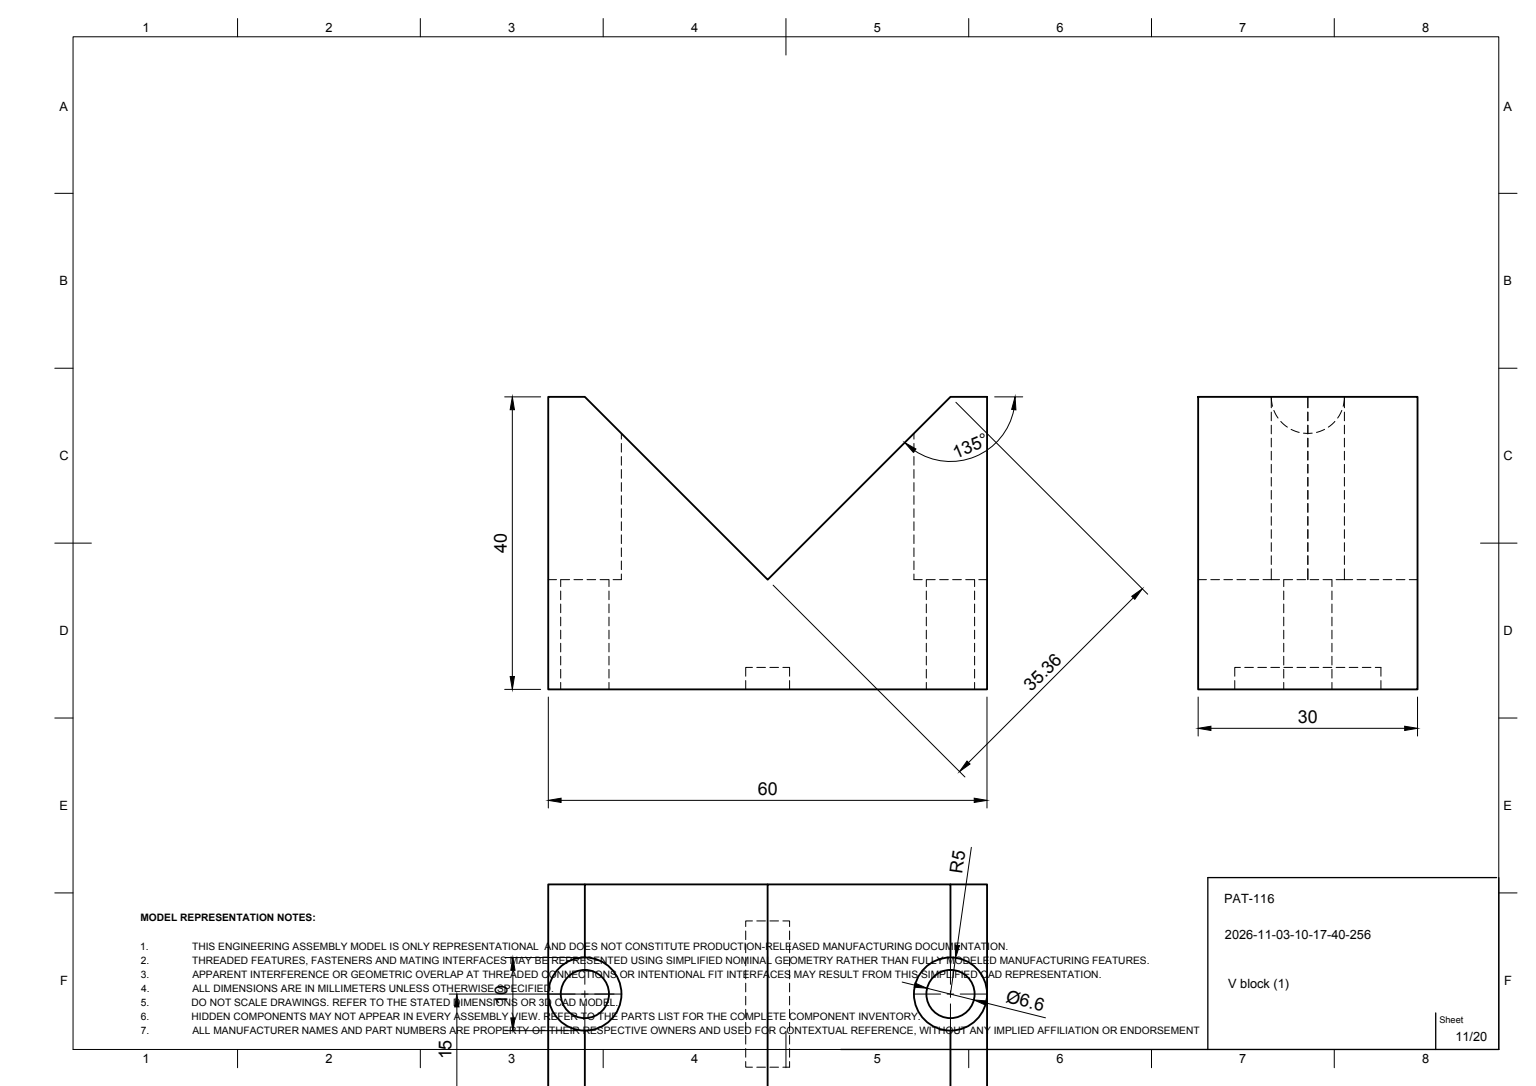
ISO-10303-21;
HEADER;
/* Generated by software containing ST-Developer
 * from STEP Tools, Inc. (www.steptools.com) 
 */

FILE_DESCRIPTION(
/* description */ ('V-block with clamp strap'),
/* implementation_level */ '2;1');

FILE_NAME(
/* name */ 'V block (1).step',
/* time_stamp */ '2026-10-27T10:50:53-07:00',
/* author */ (''),
/* organization */ (''),
/* preprocessor_version */ 'ST-DEVELOPER v20.2',
/* originating_system */ 'Autodesk Translation Framework v15.17.0.0',
/* authorisation */ '');

FILE_SCHEMA (('AUTOMOTIVE_DESIGN { 1 0 10303 214 3 1 1 }'));
ENDSEC;

DATA;
#10=MECHANICAL_DESIGN_GEOMETRIC_PRESENTATION_REPRESENTATION('',(#272),#7344);
#222=ELLIPSE('',#4545,0.707106781186547,0.5);
#223=ELLIPSE('',#4557,0.707106781186547,0.5);
#230=SHAPE_REPRESENTATION_RELATIONSHIP('SRR','None',#7448,#251);
#251=ADVANCED_BREP_SHAPE_REPRESENTATION('',(#293),#7327);
#272=STYLED_ITEM('',(#7610),#293);
#293=MANIFOLD_SOLID_BREP('Body1',#4154);
#344=FACE_BOUND('',#930,.T.);
#345=FACE_BOUND('',#933,.T.);
#346=FACE_BOUND('',#947,.T.);
#347=FACE_BOUND('',#948,.T.);
#348=FACE_BOUND('',#949,.T.);
#420=CIRCLE('',#4540,0.5);
#421=CIRCLE('',#4541,0.5);
#422=CIRCLE('',#4543,0.5);
#423=CIRCLE('',#4544,0.5);
#424=CIRCLE('',#4552,0.5);
#425=CIRCLE('',#4553,0.5);
#426=CIRCLE('',#4555,0.33);
#427=CIRCLE('',#4558,0.5);
#428=CIRCLE('',#4559,0.5);
#429=CIRCLE('',#4561,0.33);
#430=CIRCLE('',#4567,0.33);
#431=CIRCLE('',#4569,0.33);
#527=CYLINDRICAL_SURFACE('',#4539,0.5);
#528=CYLINDRICAL_SURFACE('',#4542,0.5);
#529=CYLINDRICAL_SURFACE('',#4551,0.5);
#530=CYLINDRICAL_SURFACE('',#4556,0.5);
#531=CYLINDRICAL_SURFACE('',#4566,0.33);
#532=CYLINDRICAL_SURFACE('',#4568,0.33);
#642=FACE_OUTER_BOUND('',#921,.T.);
#643=FACE_OUTER_BOUND('',#922,.T.);
#644=FACE_OUTER_BOUND('',#923,.T.);
#645=FACE_OUTER_BOUND('',#924,.T.);
#646=FACE_OUTER_BOUND('',#925,.T.);
#647=FACE_OUTER_BOUND('',#926,.T.);
#648=FACE_OUTER_BOUND('',#927,.T.);
#649=FACE_OUTER_BOUND('',#928,.T.);
#650=FACE_OUTER_BOUND('',#929,.T.);
#651=FACE_OUTER_BOUND('',#931,.T.);
#652=FACE_OUTER_BOUND('',#932,.T.);
#653=FACE_OUTER_BOUND('',#934,.T.);
#654=FACE_OUTER_BOUND('',#935,.T.);
#655=FACE_OUTER_BOUND('',#936,.T.);
#656=FACE_OUTER_BOUND('',#937,.T.);
#657=FACE_OUTER_BOUND('',#938,.T.);
#658=FACE_OUTER_BOUND('',#939,.T.);
#659=FACE_OUTER_BOUND('',#940,.T.);
#660=FACE_OUTER_BOUND('',#941,.T.);
#661=FACE_OUTER_BOUND('',#942,.T.);
#662=FACE_OUTER_BOUND('',#943,.T.);
#663=FACE_OUTER_BOUND('',#944,.T.);
#664=FACE_OUTER_BOUND('',#945,.T.);
#665=FACE_OUTER_BOUND('',#946,.T.);
#921=EDGE_LOOP('',(#3078,#3079,#3080,#3081));
#922=EDGE_LOOP('',(#3082,#3083,#3084,#3085,#3086));
#923=EDGE_LOOP('',(#3087,#3088,#3089,#3090));
#924=EDGE_LOOP('',(#3091,#3092,#3093,#3094));
#925=EDGE_LOOP('',(#3095,#3096,#3097,#3098));
#926=EDGE_LOOP('',(#3099,#3100,#3101,#3102));
#927=EDGE_LOOP('',(#3103,#3104,#3105,#3106));
#928=EDGE_LOOP('',(#3107,#3108,#3109,#3110));
#929=EDGE_LOOP('',(#3111,#3112));
#930=EDGE_LOOP('',(#3113));
#931=EDGE_LOOP('',(#3114,#3115,#3116,#3117,#3118));
#932=EDGE_LOOP('',(#3119,#3120));
#933=EDGE_LOOP('',(#3121));
#934=EDGE_LOOP('',(#3122,#3123,#3124,#3125,#3126,#3127));
#935=EDGE_LOOP('',(#3128,#3129,#3130,#3131));
#936=EDGE_LOOP('',(#3132,#3133,#3134,#3135,#3136,#3137));
#937=EDGE_LOOP('',(#3138,#3139,#3140,#3141));
#938=EDGE_LOOP('',(#3142,#3143,#3144,#3145));
#939=EDGE_LOOP('',(#3146,#3147,#3148,#3149));
#940=EDGE_LOOP('',(#3150,#3151,#3152,#3153));
#941=EDGE_LOOP('',(#3154,#3155,#3156,#3157));
#942=EDGE_LOOP('',(#3158,#3159,#3160,#3161,#3162,#3163,#3164));
#943=EDGE_LOOP('',(#3165,#3166,#3167,#3168,#3169,#3170,#3171));
#944=EDGE_LOOP('',(#3172,#3173,#3174,#3175,#3176,#3177,#3178));
#945=EDGE_LOOP('',(#3179,#3180,#3181,#3182,#3183,#3184,#3185));
#946=EDGE_LOOP('',(#3186,#3187,#3188,#3189));
#947=EDGE_LOOP('',(#3190,#3191,#3192,#3193));
#948=EDGE_LOOP('',(#3194));
#949=EDGE_LOOP('',(#3195));
#1258=LINE('',#6493,#1623);
#1259=LINE('',#6497,#1624);
#1260=LINE('',#6502,#1625);
#1261=LINE('',#6506,#1626);
#1262=LINE('',#6513,#1627);
#1263=LINE('',#6515,#1628);
#1264=LINE('',#6517,#1629);
#1265=LINE('',#6518,#1630);
#1266=LINE('',#6521,#1631);
#1267=LINE('',#6523,#1632);
#1268=LINE('',#6524,#1633);
#1269=LINE('',#6527,#1634);
#1270=LINE('',#6529,#1635);
#1271=LINE('',#6530,#1636);
#1272=LINE('',#6532,#1637);
#1273=LINE('',#6533,#1638);
#1274=LINE('',#6537,#1639);
#1275=LINE('',#6546,#1640);
#1276=LINE('',#6553,#1641);
#1277=LINE('',#6555,#1642);
#1278=LINE('',#6557,#1643);
#1279=LINE('',#6559,#1644);
#1280=LINE('',#6560,#1645);
#1281=LINE('',#6563,#1646);
#1282=LINE('',#6564,#1647);
#1283=LINE('',#6567,#1648);
#1284=LINE('',#6568,#1649);
#1285=LINE('',#6570,#1650);
#1286=LINE('',#6571,#1651);
#1287=LINE('',#6574,#1652);
#1288=LINE('',#6575,#1653);
#1289=LINE('',#6579,#1654);
#1290=LINE('',#6583,#1655);
#1291=LINE('',#6586,#1656);
#1292=LINE('',#6587,#1657);
#1293=LINE('',#6590,#1658);
#1294=LINE('',#6591,#1659);
#1295=LINE('',#6594,#1660);
#1296=LINE('',#6596,#1661);
#1297=LINE('',#6597,#1662);
#1298=LINE('',#6600,#1663);
#1299=LINE('',#6601,#1664);
#1300=LINE('',#6604,#1665);
#1301=LINE('',#6605,#1666);
#1302=LINE('',#6607,#1667);
#1623=VECTOR('',#5260,0.5);
#1624=VECTOR('',#5263,1.);
#1625=VECTOR('',#5268,0.5);
#1626=VECTOR('',#5271,1.);
#1627=VECTOR('',#5278,1.);
#1628=VECTOR('',#5279,1.);
#1629=VECTOR('',#5280,1.);
#1630=VECTOR('',#5281,1.);
#1631=VECTOR('',#5284,1.);
#1632=VECTOR('',#5285,1.);
#1633=VECTOR('',#5286,1.);
#1634=VECTOR('',#5289,1.);
#1635=VECTOR('',#5290,1.);
#1636=VECTOR('',#5291,1.);
#1637=VECTOR('',#5294,1.);
#1638=VECTOR('',#5295,1.);
#1639=VECTOR('',#5302,1.);
#1640=VECTOR('',#5315,1.);
#1641=VECTOR('',#5324,1.);
#1642=VECTOR('',#5325,1.);
#1643=VECTOR('',#5326,1.);
#1644=VECTOR('',#5327,1.);
#1645=VECTOR('',#5328,1.);
#1646=VECTOR('',#5331,1.);
#1647=VECTOR('',#5332,1.);
#1648=VECTOR('',#5335,1.);
#1649=VECTOR('',#5336,1.);
#1650=VECTOR('',#5337,1.);
#1651=VECTOR('',#5338,1.);
#1652=VECTOR('',#5341,1.);
#1653=VECTOR('',#5342,1.);
#1654=VECTOR('',#5347,0.33);
#1655=VECTOR('',#5352,0.33);
#1656=VECTOR('',#5355,1.);
#1657=VECTOR('',#5356,1.);
#1658=VECTOR('',#5359,1.);
#1659=VECTOR('',#5360,1.);
#1660=VECTOR('',#5363,1.);
#1661=VECTOR('',#5364,1.);
#1662=VECTOR('',#5365,1.);
#1663=VECTOR('',#5368,1.);
#1664=VECTOR('',#5369,1.);
#1665=VECTOR('',#5372,1.);
#1666=VECTOR('',#5373,1.);
#1667=VECTOR('',#5376,1.);
#1967=VERTEX_POINT('',#6491);
#1968=VERTEX_POINT('',#6492);
#1969=VERTEX_POINT('',#6494);
#1970=VERTEX_POINT('',#6496);
#1971=VERTEX_POINT('',#6500);
#1972=VERTEX_POINT('',#6501);
#1973=VERTEX_POINT('',#6503);
#1974=VERTEX_POINT('',#6505);
#1975=VERTEX_POINT('',#6507);
#1976=VERTEX_POINT('',#6511);
#1977=VERTEX_POINT('',#6512);
#1978=VERTEX_POINT('',#6514);
#1979=VERTEX_POINT('',#6516);
#1980=VERTEX_POINT('',#6520);
#1981=VERTEX_POINT('',#6522);
#1982=VERTEX_POINT('',#6526);
#1983=VERTEX_POINT('',#6528);
#1984=VERTEX_POINT('',#6540);
#1985=VERTEX_POINT('',#6543);
#1986=VERTEX_POINT('',#6549);
#1987=VERTEX_POINT('',#6552);
#1988=VERTEX_POINT('',#6554);
#1989=VERTEX_POINT('',#6556);
#1990=VERTEX_POINT('',#6558);
#1991=VERTEX_POINT('',#6562);
#1992=VERTEX_POINT('',#6566);
#1993=VERTEX_POINT('',#6569);
#1994=VERTEX_POINT('',#6573);
#1995=VERTEX_POINT('',#6577);
#1996=VERTEX_POINT('',#6581);
#1997=VERTEX_POINT('',#6585);
#1998=VERTEX_POINT('',#6589);
#1999=VERTEX_POINT('',#6593);
#2000=VERTEX_POINT('',#6595);
#2001=VERTEX_POINT('',#6599);
#2002=VERTEX_POINT('',#6603);
#2365=EDGE_CURVE('',#1967,#1968,#1258,.T.);
#2366=EDGE_CURVE('',#1969,#1967,#420,.T.);
#2367=EDGE_CURVE('',#1969,#1970,#1259,.T.);
#2368=EDGE_CURVE('',#1968,#1970,#421,.T.);
#2369=EDGE_CURVE('',#1971,#1972,#1260,.T.);
#2370=EDGE_CURVE('',#1973,#1971,#422,.T.);
#2371=EDGE_CURVE('',#1973,#1974,#1261,.T.);
#2372=EDGE_CURVE('',#1975,#1974,#423,.T.);
#2373=EDGE_CURVE('',#1972,#1975,#222,.T.);
#2374=EDGE_CURVE('',#1976,#1977,#1262,.T.);
#2375=EDGE_CURVE('',#1976,#1978,#1263,.T.);
#2376=EDGE_CURVE('',#1978,#1979,#1264,.T.);
#2377=EDGE_CURVE('',#1977,#1979,#1265,.T.);
#2378=EDGE_CURVE('',#1977,#1980,#1266,.T.);
#2379=EDGE_CURVE('',#1979,#1981,#1267,.T.);
#2380=EDGE_CURVE('',#1980,#1981,#1268,.T.);
#2381=EDGE_CURVE('',#1980,#1982,#1269,.T.);
#2382=EDGE_CURVE('',#1981,#1983,#1270,.T.);
#2383=EDGE_CURVE('',#1982,#1983,#1271,.T.);
#2384=EDGE_CURVE('',#1982,#1976,#1272,.T.);
#2385=EDGE_CURVE('',#1983,#1978,#1273,.T.);
#2386=EDGE_CURVE('',#1974,#1972,#424,.T.);
#2387=EDGE_CURVE('',#1973,#1974,#1274,.T.);
#2388=EDGE_CURVE('',#1971,#1973,#425,.T.);
#2389=EDGE_CURVE('',#1984,#1984,#426,.T.);
#2390=EDGE_CURVE('',#1985,#1968,#223,.T.);
#2391=EDGE_CURVE('',#1970,#1985,#427,.T.);
#2392=EDGE_CURVE('',#1969,#1970,#1275,.T.);
#2393=EDGE_CURVE('',#1967,#1969,#428,.T.);
#2394=EDGE_CURVE('',#1986,#1986,#429,.T.);
#2395=EDGE_CURVE('',#1987,#1975,#1276,.T.);
#2396=EDGE_CURVE('',#1988,#1987,#1277,.T.);
#2397=EDGE_CURVE('',#1989,#1988,#1278,.T.);
#2398=EDGE_CURVE('',#1990,#1989,#1279,.T.);
#2399=EDGE_CURVE('',#1972,#1990,#1280,.T.);
#2400=EDGE_CURVE('',#1974,#1991,#1281,.T.);
#2401=EDGE_CURVE('',#1991,#1987,#1282,.T.);
#2402=EDGE_CURVE('',#1992,#1968,#1283,.T.);
#2403=EDGE_CURVE('',#1989,#1992,#1284,.T.);
#2404=EDGE_CURVE('',#1993,#1988,#1285,.T.);
#2405=EDGE_CURVE('',#1985,#1993,#1286,.T.);
#2406=EDGE_CURVE('',#1970,#1994,#1287,.T.);
#2407=EDGE_CURVE('',#1994,#1992,#1288,.T.);
#2408=EDGE_CURVE('',#1995,#1995,#430,.T.);
#2409=EDGE_CURVE('',#1995,#1984,#1289,.T.);
#2410=EDGE_CURVE('',#1996,#1996,#431,.T.);
#2411=EDGE_CURVE('',#1996,#1986,#1290,.T.);
#2412=EDGE_CURVE('',#1990,#1997,#1291,.T.);
#2413=EDGE_CURVE('',#1997,#1974,#1292,.T.);
#2414=EDGE_CURVE('',#1993,#1998,#1293,.T.);
#2415=EDGE_CURVE('',#1998,#1970,#1294,.T.);
#2416=EDGE_CURVE('',#1999,#1994,#1295,.T.);
#2417=EDGE_CURVE('',#1999,#2000,#1296,.T.);
#2418=EDGE_CURVE('',#2000,#1997,#1297,.T.);
#2419=EDGE_CURVE('',#2001,#1999,#1298,.T.);
#2420=EDGE_CURVE('',#2001,#1998,#1299,.T.);
#2421=EDGE_CURVE('',#2002,#1991,#1300,.T.);
#2422=EDGE_CURVE('',#2002,#2001,#1301,.T.);
#2423=EDGE_CURVE('',#2000,#2002,#1302,.T.);
#3078=ORIENTED_EDGE('',*,*,#2365,.F.);
#3079=ORIENTED_EDGE('',*,*,#2366,.F.);
#3080=ORIENTED_EDGE('',*,*,#2367,.T.);
#3081=ORIENTED_EDGE('',*,*,#2368,.F.);
#3082=ORIENTED_EDGE('',*,*,#2369,.F.);
#3083=ORIENTED_EDGE('',*,*,#2370,.F.);
#3084=ORIENTED_EDGE('',*,*,#2371,.T.);
#3085=ORIENTED_EDGE('',*,*,#2372,.F.);
#3086=ORIENTED_EDGE('',*,*,#2373,.F.);
#3087=ORIENTED_EDGE('',*,*,#2374,.F.);
#3088=ORIENTED_EDGE('',*,*,#2375,.T.);
#3089=ORIENTED_EDGE('',*,*,#2376,.T.);
#3090=ORIENTED_EDGE('',*,*,#2377,.F.);
#3091=ORIENTED_EDGE('',*,*,#2378,.F.);
#3092=ORIENTED_EDGE('',*,*,#2377,.T.);
#3093=ORIENTED_EDGE('',*,*,#2379,.T.);
#3094=ORIENTED_EDGE('',*,*,#2380,.F.);
#3095=ORIENTED_EDGE('',*,*,#2381,.F.);
#3096=ORIENTED_EDGE('',*,*,#2380,.T.);
#3097=ORIENTED_EDGE('',*,*,#2382,.T.);
#3098=ORIENTED_EDGE('',*,*,#2383,.F.);
#3099=ORIENTED_EDGE('',*,*,#2384,.F.);
#3100=ORIENTED_EDGE('',*,*,#2383,.T.);
#3101=ORIENTED_EDGE('',*,*,#2385,.T.);
#3102=ORIENTED_EDGE('',*,*,#2375,.F.);
#3103=ORIENTED_EDGE('',*,*,#2385,.F.);
#3104=ORIENTED_EDGE('',*,*,#2382,.F.);
#3105=ORIENTED_EDGE('',*,*,#2379,.F.);
#3106=ORIENTED_EDGE('',*,*,#2376,.F.);
#3107=ORIENTED_EDGE('',*,*,#2369,.T.);
#3108=ORIENTED_EDGE('',*,*,#2386,.F.);
#3109=ORIENTED_EDGE('',*,*,#2387,.F.);
#3110=ORIENTED_EDGE('',*,*,#2388,.F.);
#3111=ORIENTED_EDGE('',*,*,#2370,.T.);
#3112=ORIENTED_EDGE('',*,*,#2388,.T.);
#3113=ORIENTED_EDGE('',*,*,#2389,.F.);
#3114=ORIENTED_EDGE('',*,*,#2365,.T.);
#3115=ORIENTED_EDGE('',*,*,#2390,.F.);
#3116=ORIENTED_EDGE('',*,*,#2391,.F.);
#3117=ORIENTED_EDGE('',*,*,#2392,.F.);
#3118=ORIENTED_EDGE('',*,*,#2393,.F.);
#3119=ORIENTED_EDGE('',*,*,#2366,.T.);
#3120=ORIENTED_EDGE('',*,*,#2393,.T.);
#3121=ORIENTED_EDGE('',*,*,#2394,.F.);
#3122=ORIENTED_EDGE('',*,*,#2373,.T.);
#3123=ORIENTED_EDGE('',*,*,#2395,.F.);
#3124=ORIENTED_EDGE('',*,*,#2396,.F.);
#3125=ORIENTED_EDGE('',*,*,#2397,.F.);
#3126=ORIENTED_EDGE('',*,*,#2398,.F.);
#3127=ORIENTED_EDGE('',*,*,#2399,.F.);
#3128=ORIENTED_EDGE('',*,*,#2372,.T.);
#3129=ORIENTED_EDGE('',*,*,#2400,.T.);
#3130=ORIENTED_EDGE('',*,*,#2401,.T.);
#3131=ORIENTED_EDGE('',*,*,#2395,.T.);
#3132=ORIENTED_EDGE('',*,*,#2390,.T.);
#3133=ORIENTED_EDGE('',*,*,#2402,.F.);
#3134=ORIENTED_EDGE('',*,*,#2403,.F.);
#3135=ORIENTED_EDGE('',*,*,#2397,.T.);
#3136=ORIENTED_EDGE('',*,*,#2404,.F.);
#3137=ORIENTED_EDGE('',*,*,#2405,.F.);
#3138=ORIENTED_EDGE('',*,*,#2368,.T.);
#3139=ORIENTED_EDGE('',*,*,#2406,.T.);
#3140=ORIENTED_EDGE('',*,*,#2407,.T.);
#3141=ORIENTED_EDGE('',*,*,#2402,.T.);
#3142=ORIENTED_EDGE('',*,*,#2408,.F.);
#3143=ORIENTED_EDGE('',*,*,#2409,.T.);
#3144=ORIENTED_EDGE('',*,*,#2389,.T.);
#3145=ORIENTED_EDGE('',*,*,#2409,.F.);
#3146=ORIENTED_EDGE('',*,*,#2410,.F.);
#3147=ORIENTED_EDGE('',*,*,#2411,.T.);
#3148=ORIENTED_EDGE('',*,*,#2394,.T.);
#3149=ORIENTED_EDGE('',*,*,#2411,.F.);
#3150=ORIENTED_EDGE('',*,*,#2386,.T.);
#3151=ORIENTED_EDGE('',*,*,#2399,.T.);
#3152=ORIENTED_EDGE('',*,*,#2412,.T.);
#3153=ORIENTED_EDGE('',*,*,#2413,.T.);
#3154=ORIENTED_EDGE('',*,*,#2391,.T.);
#3155=ORIENTED_EDGE('',*,*,#2405,.T.);
#3156=ORIENTED_EDGE('',*,*,#2414,.T.);
#3157=ORIENTED_EDGE('',*,*,#2415,.T.);
#3158=ORIENTED_EDGE('',*,*,#2398,.T.);
#3159=ORIENTED_EDGE('',*,*,#2403,.T.);
#3160=ORIENTED_EDGE('',*,*,#2407,.F.);
#3161=ORIENTED_EDGE('',*,*,#2416,.F.);
#3162=ORIENTED_EDGE('',*,*,#2417,.T.);
#3163=ORIENTED_EDGE('',*,*,#2418,.T.);
#3164=ORIENTED_EDGE('',*,*,#2412,.F.);
#3165=ORIENTED_EDGE('',*,*,#2419,.T.);
#3166=ORIENTED_EDGE('',*,*,#2416,.T.);
#3167=ORIENTED_EDGE('',*,*,#2406,.F.);
#3168=ORIENTED_EDGE('',*,*,#2367,.F.);
#3169=ORIENTED_EDGE('',*,*,#2392,.T.);
#3170=ORIENTED_EDGE('',*,*,#2415,.F.);
#3171=ORIENTED_EDGE('',*,*,#2420,.F.);
#3172=ORIENTED_EDGE('',*,*,#2396,.T.);
#3173=ORIENTED_EDGE('',*,*,#2401,.F.);
#3174=ORIENTED_EDGE('',*,*,#2421,.F.);
#3175=ORIENTED_EDGE('',*,*,#2422,.T.);
#3176=ORIENTED_EDGE('',*,*,#2420,.T.);
#3177=ORIENTED_EDGE('',*,*,#2414,.F.);
#3178=ORIENTED_EDGE('',*,*,#2404,.T.);
#3179=ORIENTED_EDGE('',*,*,#2423,.T.);
#3180=ORIENTED_EDGE('',*,*,#2421,.T.);
#3181=ORIENTED_EDGE('',*,*,#2400,.F.);
#3182=ORIENTED_EDGE('',*,*,#2371,.F.);
#3183=ORIENTED_EDGE('',*,*,#2387,.T.);
#3184=ORIENTED_EDGE('',*,*,#2413,.F.);
#3185=ORIENTED_EDGE('',*,*,#2418,.F.);
#3186=ORIENTED_EDGE('',*,*,#2417,.F.);
#3187=ORIENTED_EDGE('',*,*,#2419,.F.);
#3188=ORIENTED_EDGE('',*,*,#2422,.F.);
#3189=ORIENTED_EDGE('',*,*,#2423,.F.);
#3190=ORIENTED_EDGE('',*,*,#2381,.T.);
#3191=ORIENTED_EDGE('',*,*,#2384,.T.);
#3192=ORIENTED_EDGE('',*,*,#2374,.T.);
#3193=ORIENTED_EDGE('',*,*,#2378,.T.);
#3194=ORIENTED_EDGE('',*,*,#2408,.T.);
#3195=ORIENTED_EDGE('',*,*,#2410,.T.);
#3798=PLANE('',#4546);
#3799=PLANE('',#4547);
#3800=PLANE('',#4548);
#3801=PLANE('',#4549);
#3802=PLANE('',#4550);
#3803=PLANE('',#4554);
#3804=PLANE('',#4560);
#3805=PLANE('',#4562);
#3806=PLANE('',#4563);
#3807=PLANE('',#4564);
#3808=PLANE('',#4565);
#3809=PLANE('',#4570);
#3810=PLANE('',#4571);
#3811=PLANE('',#4572);
#3812=PLANE('',#4573);
#3813=PLANE('',#4574);
#3814=PLANE('',#4575);
#3815=PLANE('',#4576);
#3988=ADVANCED_FACE('',(#642),#527,.F.);
#3989=ADVANCED_FACE('',(#643),#528,.F.);
#3990=ADVANCED_FACE('',(#644),#3798,.F.);
#3991=ADVANCED_FACE('',(#645),#3799,.F.);
#3992=ADVANCED_FACE('',(#646),#3800,.F.);
#3993=ADVANCED_FACE('',(#647),#3801,.F.);
#3994=ADVANCED_FACE('',(#648),#3802,.F.);
#3995=ADVANCED_FACE('',(#649),#529,.F.);
#3996=ADVANCED_FACE('',(#650,#344),#3803,.T.);
#3997=ADVANCED_FACE('',(#651),#530,.F.);
#3998=ADVANCED_FACE('',(#652,#345),#3804,.T.);
#3999=ADVANCED_FACE('',(#653),#3805,.F.);
#4000=ADVANCED_FACE('',(#654),#3806,.T.);
#4001=ADVANCED_FACE('',(#655),#3807,.F.);
#4002=ADVANCED_FACE('',(#656),#3808,.T.);
#4003=ADVANCED_FACE('',(#657),#531,.F.);
#4004=ADVANCED_FACE('',(#658),#532,.F.);
#4005=ADVANCED_FACE('',(#659),#3809,.T.);
#4006=ADVANCED_FACE('',(#660),#3810,.T.);
#4007=ADVANCED_FACE('',(#661),#3811,.T.);
#4008=ADVANCED_FACE('',(#662),#3812,.T.);
#4009=ADVANCED_FACE('',(#663),#3813,.T.);
#4010=ADVANCED_FACE('',(#664),#3814,.T.);
#4011=ADVANCED_FACE('',(#665,#346,#347,#348),#3815,.F.);
#4154=CLOSED_SHELL('',(#3988,#3989,#3990,#3991,#3992,#3993,#3994,#3995,
#3996,#3997,#3998,#3999,#4000,#4001,#4002,#4003,#4004,#4005,#4006,#4007,
#4008,#4009,#4010,#4011));
#4538=AXIS2_PLACEMENT_3D('',#6489,#5256,#5257);
#4539=AXIS2_PLACEMENT_3D('',#6490,#5258,#5259);
#4540=AXIS2_PLACEMENT_3D('',#6495,#5261,#5262);
#4541=AXIS2_PLACEMENT_3D('',#6498,#5264,#5265);
#4542=AXIS2_PLACEMENT_3D('',#6499,#5266,#5267);
#4543=AXIS2_PLACEMENT_3D('',#6504,#5269,#5270);
#4544=AXIS2_PLACEMENT_3D('',#6508,#5272,#5273);
#4545=AXIS2_PLACEMENT_3D('',#6509,#5274,#5275);
#4546=AXIS2_PLACEMENT_3D('',#6510,#5276,#5277);
#4547=AXIS2_PLACEMENT_3D('',#6519,#5282,#5283);
#4548=AXIS2_PLACEMENT_3D('',#6525,#5287,#5288);
#4549=AXIS2_PLACEMENT_3D('',#6531,#5292,#5293);
#4550=AXIS2_PLACEMENT_3D('',#6534,#5296,#5297);
#4551=AXIS2_PLACEMENT_3D('',#6535,#5298,#5299);
#4552=AXIS2_PLACEMENT_3D('',#6536,#5300,#5301);
#4553=AXIS2_PLACEMENT_3D('',#6538,#5303,#5304);
#4554=AXIS2_PLACEMENT_3D('',#6539,#5305,#5306);
#4555=AXIS2_PLACEMENT_3D('',#6541,#5307,#5308);
#4556=AXIS2_PLACEMENT_3D('',#6542,#5309,#5310);
#4557=AXIS2_PLACEMENT_3D('',#6544,#5311,#5312);
#4558=AXIS2_PLACEMENT_3D('',#6545,#5313,#5314);
#4559=AXIS2_PLACEMENT_3D('',#6547,#5316,#5317);
#4560=AXIS2_PLACEMENT_3D('',#6548,#5318,#5319);
#4561=AXIS2_PLACEMENT_3D('',#6550,#5320,#5321);
#4562=AXIS2_PLACEMENT_3D('',#6551,#5322,#5323);
#4563=AXIS2_PLACEMENT_3D('',#6561,#5329,#5330);
#4564=AXIS2_PLACEMENT_3D('',#6565,#5333,#5334);
#4565=AXIS2_PLACEMENT_3D('',#6572,#5339,#5340);
#4566=AXIS2_PLACEMENT_3D('',#6576,#5343,#5344);
#4567=AXIS2_PLACEMENT_3D('',#6578,#5345,#5346);
#4568=AXIS2_PLACEMENT_3D('',#6580,#5348,#5349);
#4569=AXIS2_PLACEMENT_3D('',#6582,#5350,#5351);
#4570=AXIS2_PLACEMENT_3D('',#6584,#5353,#5354);
#4571=AXIS2_PLACEMENT_3D('',#6588,#5357,#5358);
#4572=AXIS2_PLACEMENT_3D('',#6592,#5361,#5362);
#4573=AXIS2_PLACEMENT_3D('',#6598,#5366,#5367);
#4574=AXIS2_PLACEMENT_3D('',#6602,#5370,#5371);
#4575=AXIS2_PLACEMENT_3D('',#6606,#5374,#5375);
#4576=AXIS2_PLACEMENT_3D('',#6608,#5377,#5378);
#5256=DIRECTION('axis',(0.,0.,1.));
#5257=DIRECTION('refdir',(1.,0.,0.));
#5258=DIRECTION('center_axis',(0.,0.,1.));
#5259=DIRECTION('ref_axis',(1.,0.,0.));
#5260=DIRECTION('',(0.,0.,1.));
#5261=DIRECTION('center_axis',(0.,0.,1.));
#5262=DIRECTION('ref_axis',(1.,0.,0.));
#5263=DIRECTION('',(0.,0.,1.));
#5264=DIRECTION('center_axis',(0.,0.,-1.));
#5265=DIRECTION('ref_axis',(1.,0.,0.));
#5266=DIRECTION('center_axis',(0.,0.,1.));
#5267=DIRECTION('ref_axis',(1.,0.,0.));
#5268=DIRECTION('',(0.,0.,1.));
#5269=DIRECTION('center_axis',(0.,0.,1.));
#5270=DIRECTION('ref_axis',(1.,0.,0.));
#5271=DIRECTION('',(0.,0.,1.));
#5272=DIRECTION('center_axis',(0.,0.,-1.));
#5273=DIRECTION('ref_axis',(1.,0.,0.));
#5274=DIRECTION('center_axis',(0.,-0.707106781186547,-0.707106781186548));
#5275=DIRECTION('ref_axis',(0.,0.707106781186548,-0.707106781186547));
#5276=DIRECTION('center_axis',(0.,-1.,0.));
#5277=DIRECTION('ref_axis',(1.,0.,0.));
#5278=DIRECTION('',(1.,0.,0.));
#5279=DIRECTION('',(0.,0.,1.));
#5280=DIRECTION('',(1.,0.,0.));
#5281=DIRECTION('',(0.,0.,1.));
#5282=DIRECTION('center_axis',(1.,0.,0.));
#5283=DIRECTION('ref_axis',(0.,1.,0.));
#5284=DIRECTION('',(0.,1.,0.));
#5285=DIRECTION('',(0.,1.,0.));
#5286=DIRECTION('',(0.,0.,1.));
#5287=DIRECTION('center_axis',(0.,1.,0.));
#5288=DIRECTION('ref_axis',(-1.,0.,0.));
#5289=DIRECTION('',(-1.,0.,0.));
#5290=DIRECTION('',(-1.,0.,0.));
#5291=DIRECTION('',(0.,0.,1.));
#5292=DIRECTION('center_axis',(-1.,0.,0.));
#5293=DIRECTION('ref_axis',(0.,-1.,0.));
#5294=DIRECTION('',(0.,-1.,0.));
#5295=DIRECTION('',(0.,-1.,0.));
#5296=DIRECTION('center_axis',(0.,0.,1.));
#5297=DIRECTION('ref_axis',(1.,0.,0.));
#5298=DIRECTION('center_axis',(0.,0.,1.));
#5299=DIRECTION('ref_axis',(1.,0.,0.));
#5300=DIRECTION('center_axis',(0.,0.,-1.));
#5301=DIRECTION('ref_axis',(1.,0.,0.));
#5302=DIRECTION('',(0.,0.,1.));
#5303=DIRECTION('center_axis',(0.,0.,1.));
#5304=DIRECTION('ref_axis',(1.,0.,0.));
#5305=DIRECTION('center_axis',(0.,0.,1.));
#5306=DIRECTION('ref_axis',(1.,0.,0.));
#5307=DIRECTION('center_axis',(0.,0.,1.));
#5308=DIRECTION('ref_axis',(1.,0.,0.));
#5309=DIRECTION('center_axis',(0.,0.,1.));
#5310=DIRECTION('ref_axis',(1.,0.,0.));
#5311=DIRECTION('center_axis',(0.,0.707106781186547,-0.707106781186548));
#5312=DIRECTION('ref_axis',(0.,0.707106781186548,0.707106781186547));
#5313=DIRECTION('center_axis',(0.,0.,-1.));
#5314=DIRECTION('ref_axis',(1.,0.,0.));
#5315=DIRECTION('',(0.,0.,1.));
#5316=DIRECTION('center_axis',(0.,0.,1.));
#5317=DIRECTION('ref_axis',(1.,0.,0.));
#5318=DIRECTION('center_axis',(0.,0.,1.));
#5319=DIRECTION('ref_axis',(1.,0.,0.));
#5320=DIRECTION('center_axis',(0.,0.,1.));
#5321=DIRECTION('ref_axis',(1.,0.,0.));
#5322=DIRECTION('center_axis',(0.,-0.707106781186547,-0.707106781186548));
#5323=DIRECTION('ref_axis',(0.,0.707106781186548,-0.707106781186547));
#5324=DIRECTION('',(-1.,0.,0.));
#5325=DIRECTION('',(0.,-0.707106781186548,0.707106781186547));
#5326=DIRECTION('',(1.,0.,0.));
#5327=DIRECTION('',(0.,0.707106781186548,-0.707106781186547));
#5328=DIRECTION('',(-1.,0.,0.));
#5329=DIRECTION('center_axis',(0.,0.,1.));
#5330=DIRECTION('ref_axis',(1.,0.,0.));
#5331=DIRECTION('',(1.,0.,0.));
#5332=DIRECTION('',(0.,1.,0.));
#5333=DIRECTION('center_axis',(0.,0.707106781186547,-0.707106781186548));
#5334=DIRECTION('ref_axis',(0.,0.707106781186548,0.707106781186547));
#5335=DIRECTION('',(1.,0.,0.));
#5336=DIRECTION('',(0.,0.707106781186548,0.707106781186547));
#5337=DIRECTION('',(0.,-0.707106781186548,-0.707106781186547));
#5338=DIRECTION('',(1.,0.,0.));
#5339=DIRECTION('center_axis',(0.,0.,1.));
#5340=DIRECTION('ref_axis',(1.,0.,0.));
#5341=DIRECTION('',(-1.,0.,0.));
#5342=DIRECTION('',(0.,-1.,0.));
#5343=DIRECTION('center_axis',(0.,0.,1.));
#5344=DIRECTION('ref_axis',(1.,0.,0.));
#5345=DIRECTION('center_axis',(0.,0.,1.));
#5346=DIRECTION('ref_axis',(1.,0.,0.));
#5347=DIRECTION('',(0.,0.,1.));
#5348=DIRECTION('center_axis',(0.,0.,1.));
#5349=DIRECTION('ref_axis',(1.,0.,0.));
#5350=DIRECTION('center_axis',(0.,0.,1.));
#5351=DIRECTION('ref_axis',(1.,0.,0.));
#5352=DIRECTION('',(0.,0.,1.));
#5353=DIRECTION('center_axis',(0.,0.,1.));
#5354=DIRECTION('ref_axis',(1.,0.,0.));
#5355=DIRECTION('',(0.,-1.,0.));
#5356=DIRECTION('',(1.,0.,0.));
#5357=DIRECTION('center_axis',(0.,0.,1.));
#5358=DIRECTION('ref_axis',(1.,0.,0.));
#5359=DIRECTION('',(0.,1.,0.));
#5360=DIRECTION('',(-1.,0.,0.));
#5361=DIRECTION('center_axis',(-1.,0.,0.));
#5362=DIRECTION('ref_axis',(0.,-1.,0.));
#5363=DIRECTION('',(0.,0.,1.));
#5364=DIRECTION('',(0.,-1.,0.));
#5365=DIRECTION('',(0.,0.,1.));
#5366=DIRECTION('center_axis',(0.,1.,0.));
#5367=DIRECTION('ref_axis',(-1.,0.,0.));
#5368=DIRECTION('',(-1.,0.,0.));
#5369=DIRECTION('',(0.,0.,1.));
#5370=DIRECTION('center_axis',(1.,0.,0.));
#5371=DIRECTION('ref_axis',(0.,1.,0.));
#5372=DIRECTION('',(0.,0.,1.));
#5373=DIRECTION('',(0.,1.,0.));
#5374=DIRECTION('center_axis',(0.,-1.,0.));
#5375=DIRECTION('ref_axis',(1.,0.,0.));
#5376=DIRECTION('',(1.,0.,0.));
#5377=DIRECTION('center_axis',(0.,0.,1.));
#5378=DIRECTION('ref_axis',(1.,0.,0.));
#6489=CARTESIAN_POINT('',(0.,0.,0.));
#6490=CARTESIAN_POINT('Origin',(13.5,2.5,2.5));
#6491=CARTESIAN_POINT('',(13.,2.5,2.5));
#6492=CARTESIAN_POINT('',(13.,2.5,5.));
#6493=CARTESIAN_POINT('',(13.,2.5,2.5));
#6494=CARTESIAN_POINT('',(13.5,3.,2.5));
#6495=CARTESIAN_POINT('Origin',(13.5,2.5,2.5));
#6496=CARTESIAN_POINT('',(13.5,3.,5.));
#6497=CARTESIAN_POINT('',(13.5,3.,2.5));
#6498=CARTESIAN_POINT('Origin',(13.5,2.5,5.));
#6499=CARTESIAN_POINT('Origin',(13.5,-2.5,2.5));
#6500=CARTESIAN_POINT('',(13.,-2.5,2.5));
#6501=CARTESIAN_POINT('',(13.,-2.5,5.));
#6502=CARTESIAN_POINT('',(13.,-2.5,2.5));
#6503=CARTESIAN_POINT('',(13.5,-3.,2.5));
#6504=CARTESIAN_POINT('Origin',(13.5,-2.5,2.5));
#6505=CARTESIAN_POINT('',(13.5,-3.,5.));
#6506=CARTESIAN_POINT('',(13.5,-3.,2.5));
#6507=CARTESIAN_POINT('',(14.,-2.5,5.));
#6508=CARTESIAN_POINT('Origin',(13.5,-2.5,5.));
#6509=CARTESIAN_POINT('Origin',(13.5,-2.5,5.));
#6510=CARTESIAN_POINT('Origin',(12.5,-0.3,0.9));
#6511=CARTESIAN_POINT('',(12.5,-0.3,1.));
#6512=CARTESIAN_POINT('',(14.5,-0.3,1.));
#6513=CARTESIAN_POINT('',(13.,-0.3,1.));
#6514=CARTESIAN_POINT('',(12.5,-0.3,1.3));
#6515=CARTESIAN_POINT('',(12.5,-0.3,0.9));
#6516=CARTESIAN_POINT('',(14.5,-0.3,1.3));
#6517=CARTESIAN_POINT('',(12.5,-0.3,1.3));
#6518=CARTESIAN_POINT('',(14.5,-0.3,0.9));
#6519=CARTESIAN_POINT('Origin',(14.5,-0.3,0.9));
#6520=CARTESIAN_POINT('',(14.5,0.3,1.));
#6521=CARTESIAN_POINT('',(14.5,-0.15,1.));
#6522=CARTESIAN_POINT('',(14.5,0.3,1.3));
#6523=CARTESIAN_POINT('',(14.5,-0.3,1.3));
#6524=CARTESIAN_POINT('',(14.5,0.3,0.9));
#6525=CARTESIAN_POINT('Origin',(14.5,0.3,0.9));
#6526=CARTESIAN_POINT('',(12.5,0.3,1.));
#6527=CARTESIAN_POINT('',(14.,0.3,1.));
#6528=CARTESIAN_POINT('',(12.5,0.3,1.3));
#6529=CARTESIAN_POINT('',(14.5,0.3,1.3));
#6530=CARTESIAN_POINT('',(12.5,0.3,0.9));
#6531=CARTESIAN_POINT('Origin',(12.5,0.3,0.9));
#6532=CARTESIAN_POINT('',(12.5,0.15,1.));
#6533=CARTESIAN_POINT('',(12.5,0.3,1.3));
#6534=CARTESIAN_POINT('Origin',(13.5,0.,1.3));
#6535=CARTESIAN_POINT('Origin',(13.5,-2.5,2.5));
#6536=CARTESIAN_POINT('Origin',(13.5,-2.5,5.));
#6537=CARTESIAN_POINT('',(13.5,-3.,2.5));
#6538=CARTESIAN_POINT('Origin',(13.5,-2.5,2.5));
#6539=CARTESIAN_POINT('Origin',(13.5,-2.5,2.5));
#6540=CARTESIAN_POINT('',(13.17,-2.5,2.5));
#6541=CARTESIAN_POINT('Origin',(13.5,-2.5,2.5));
#6542=CARTESIAN_POINT('Origin',(13.5,2.5,2.5));
#6543=CARTESIAN_POINT('',(14.,2.5,5.));
#6544=CARTESIAN_POINT('Origin',(13.5,2.5,5.));
#6545=CARTESIAN_POINT('Origin',(13.5,2.5,5.));
#6546=CARTESIAN_POINT('',(13.5,3.,2.5));
#6547=CARTESIAN_POINT('Origin',(13.5,2.5,2.5));
#6548=CARTESIAN_POINT('Origin',(13.5,2.5,2.5));
#6549=CARTESIAN_POINT('',(13.17,2.5,2.5));
#6550=CARTESIAN_POINT('Origin',(13.5,2.5,2.5));
#6551=CARTESIAN_POINT('Origin',(11.9,-2.6,5.1));
#6552=CARTESIAN_POINT('',(15.,-2.5,5.));
#6553=CARTESIAN_POINT('',(12.7,-2.5,5.));
#6554=CARTESIAN_POINT('',(15.,0.,2.5));
#6555=CARTESIAN_POINT('',(15.,-1.675,4.175));
#6556=CARTESIAN_POINT('',(12.,0.,2.5));
#6557=CARTESIAN_POINT('',(11.9,0.,2.5));
#6558=CARTESIAN_POINT('',(12.,-2.5,5.));
#6559=CARTESIAN_POINT('',(12.,-0.175,2.675));
#6560=CARTESIAN_POINT('',(12.7,-2.5,5.));
#6561=CARTESIAN_POINT('Origin',(13.5,0.,5.));
#6562=CARTESIAN_POINT('',(15.,-3.,5.));
#6563=CARTESIAN_POINT('',(12.,-3.,5.));
#6564=CARTESIAN_POINT('',(15.,-3.,5.));
#6565=CARTESIAN_POINT('Origin',(11.9,0.,2.5));
#6566=CARTESIAN_POINT('',(12.,2.5,5.));
#6567=CARTESIAN_POINT('',(12.7,2.5,5.));
#6568=CARTESIAN_POINT('',(12.,0.375,2.875));
#6569=CARTESIAN_POINT('',(15.,2.5,5.));
#6570=CARTESIAN_POINT('',(15.,-1.125,1.375));
#6571=CARTESIAN_POINT('',(12.7,2.5,5.));
#6572=CARTESIAN_POINT('Origin',(13.5,0.,5.));
#6573=CARTESIAN_POINT('',(12.,3.,5.));
#6574=CARTESIAN_POINT('',(15.,3.,5.));
#6575=CARTESIAN_POINT('',(12.,3.,5.));
#6576=CARTESIAN_POINT('Origin',(13.5,-2.5,0.9));
#6577=CARTESIAN_POINT('',(13.17,-2.5,1.));
#6578=CARTESIAN_POINT('Origin',(13.5,-2.5,1.));
#6579=CARTESIAN_POINT('',(13.17,-2.5,0.9));
#6580=CARTESIAN_POINT('Origin',(13.5,2.5,0.9));
#6581=CARTESIAN_POINT('',(13.17,2.5,1.));
#6582=CARTESIAN_POINT('Origin',(13.5,2.5,1.));
#6583=CARTESIAN_POINT('',(13.17,2.5,0.9));
#6584=CARTESIAN_POINT('Origin',(13.5,0.,5.));
#6585=CARTESIAN_POINT('',(12.,-3.,5.));
#6586=CARTESIAN_POINT('',(12.,3.,5.));
#6587=CARTESIAN_POINT('',(12.,-3.,5.));
#6588=CARTESIAN_POINT('Origin',(13.5,0.,5.));
#6589=CARTESIAN_POINT('',(15.,3.,5.));
#6590=CARTESIAN_POINT('',(15.,-3.,5.));
#6591=CARTESIAN_POINT('',(15.,3.,5.));
#6592=CARTESIAN_POINT('Origin',(12.,3.,1.));
#6593=CARTESIAN_POINT('',(12.,3.,1.));
#6594=CARTESIAN_POINT('',(12.,3.,1.));
#6595=CARTESIAN_POINT('',(12.,-3.,1.));
#6596=CARTESIAN_POINT('',(12.,3.,1.));
#6597=CARTESIAN_POINT('',(12.,-3.,1.));
#6598=CARTESIAN_POINT('Origin',(15.,3.,1.));
#6599=CARTESIAN_POINT('',(15.,3.,1.));
#6600=CARTESIAN_POINT('',(15.,3.,1.));
#6601=CARTESIAN_POINT('',(15.,3.,1.));
#6602=CARTESIAN_POINT('Origin',(15.,-3.,1.));
#6603=CARTESIAN_POINT('',(15.,-3.,1.));
#6604=CARTESIAN_POINT('',(15.,-3.,1.));
#6605=CARTESIAN_POINT('',(15.,-3.,1.));
#6606=CARTESIAN_POINT('Origin',(12.,-3.,1.));
#6607=CARTESIAN_POINT('',(12.,-3.,1.));
#6608=CARTESIAN_POINT('Origin',(13.5,0.,1.));
#7301=UNCERTAINTY_MEASURE_WITH_UNIT(LENGTH_MEASURE(0.001),#7345,
'DISTANCE_ACCURACY_VALUE',
'Maximum model space distance between geometric entities at asserted c
onnectivities');
#7318=UNCERTAINTY_MEASURE_WITH_UNIT(LENGTH_MEASURE(0.001),#7345,
'DISTANCE_ACCURACY_VALUE',
'Maximum model space distance between geometric entities at asserted c
onnectivities');
#7327=(
GEOMETRIC_REPRESENTATION_CONTEXT(3)
GLOBAL_UNCERTAINTY_ASSIGNED_CONTEXT((#7301))
GLOBAL_UNIT_ASSIGNED_CONTEXT((#7345,#7347,#7348))
REPRESENTATION_CONTEXT('','3D')
);
#7344=(
GEOMETRIC_REPRESENTATION_CONTEXT(3)
GLOBAL_UNCERTAINTY_ASSIGNED_CONTEXT((#7318))
GLOBAL_UNIT_ASSIGNED_CONTEXT((#7345,#7347,#7348))
REPRESENTATION_CONTEXT('','3D')
);
#7345=(
LENGTH_UNIT()
NAMED_UNIT(*)
SI_UNIT(.CENTI.,.METRE.)
);
#7347=(
NAMED_UNIT(*)
PLANE_ANGLE_UNIT()
SI_UNIT($,.RADIAN.)
);
#7348=(
NAMED_UNIT(*)
SI_UNIT($,.STERADIAN.)
SOLID_ANGLE_UNIT()
);
#7357=SHAPE_DEFINITION_REPRESENTATION(#7382,#7448);
#7382=PRODUCT_DEFINITION_SHAPE('',$,#7474);
#7448=SHAPE_REPRESENTATION('',(#4538),#7327);
#7465=PRODUCT_DEFINITION_CONTEXT('part definition',#7542,'design');
#7474=PRODUCT_DEFINITION('V block (1)','V block (1)',#7499,#7465);
#7499=PRODUCT_DEFINITION_FORMATION('',$,#7552);
#7542=APPLICATION_CONTEXT(
'Core Data for Automotive Mechanical Design Process');
#7543=PRODUCT_CONTEXT('part definition',#7542,'mechanical');
#7552=PRODUCT('V block (1)','V block (1)','V block (1)',(#7543));
#7604=COLOUR_RGB('Dark Blue',0.08,0.2,0.34);
#7605=FILL_AREA_STYLE_COLOUR('',#7604);
#7606=FILL_AREA_STYLE('',(#7605));
#7607=SURFACE_STYLE_FILL_AREA(#7606);
#7608=SURFACE_SIDE_STYLE('',(#7607));
#7609=SURFACE_STYLE_USAGE(.BOTH.,#7608);
#7610=PRESENTATION_STYLE_ASSIGNMENT((#7609));
ENDSEC;
END-ISO-10303-21;
